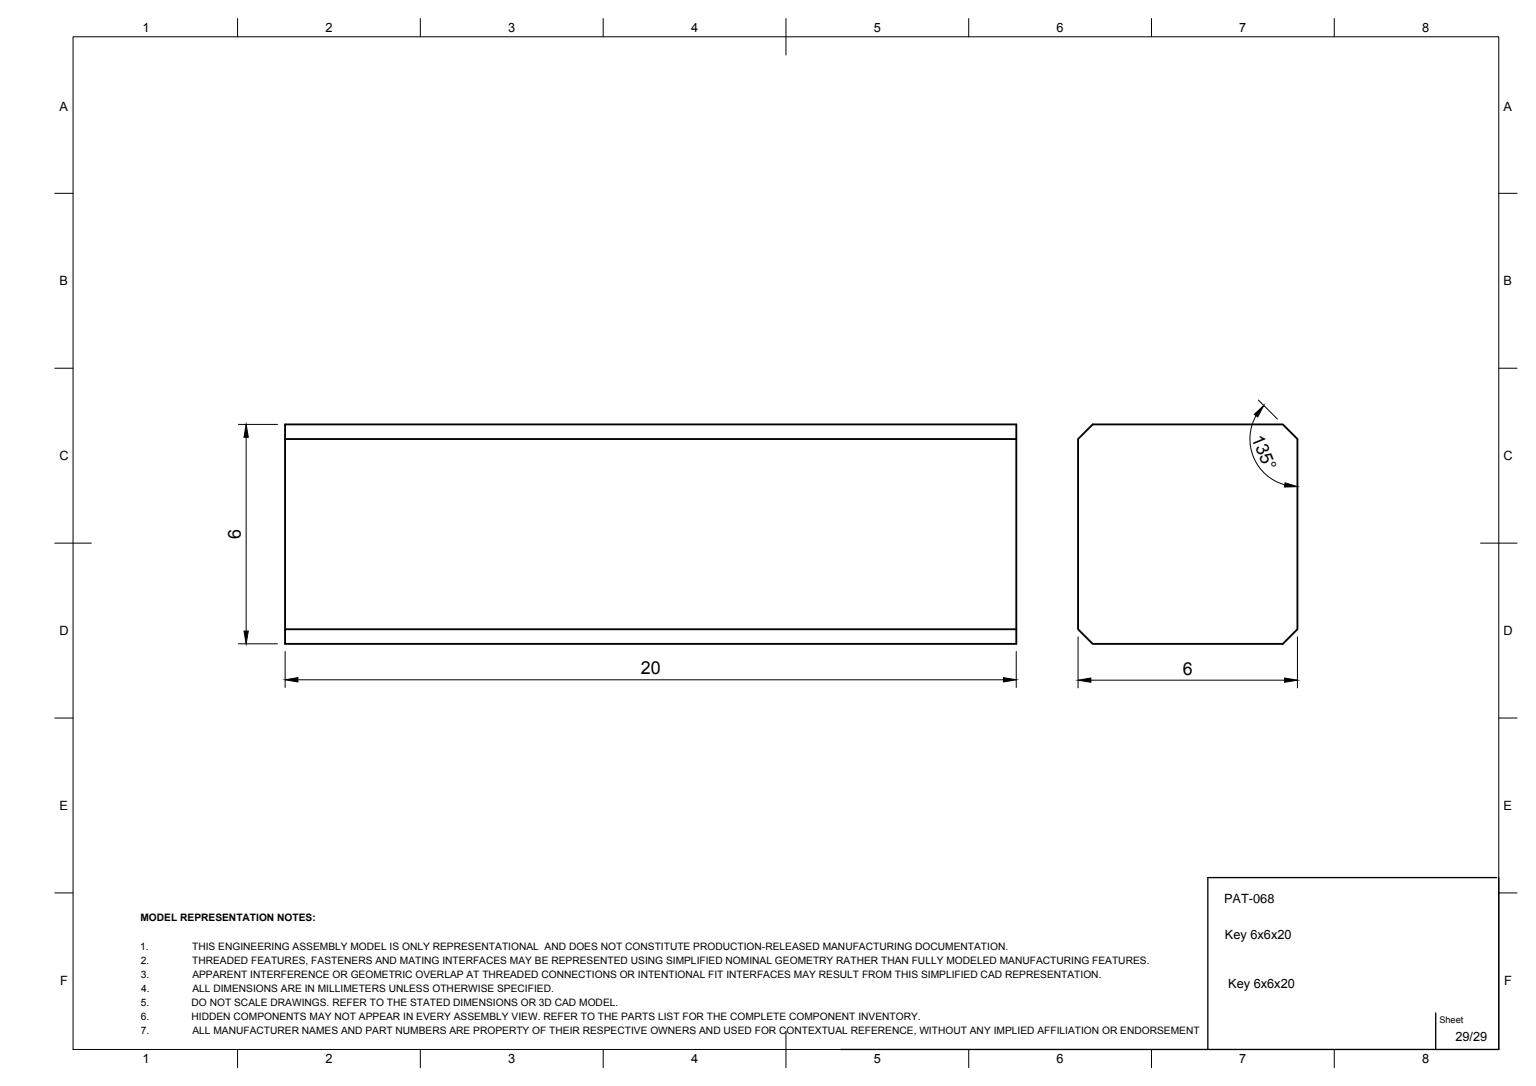
ISO-10303-21;
HEADER;
/* Generated by software containing ST-Developer
 * from STEP Tools, Inc. (www.steptools.com) 
 */

FILE_DESCRIPTION(
/* description */ ('Line shaft on three pillow blocks'),
/* implementation_level */ '2;1');

FILE_NAME(
/* name */ 'Key 6x6x20.step',
/* time_stamp */ '2026-10-27T10:49:19-07:00',
/* author */ (''),
/* organization */ (''),
/* preprocessor_version */ 'ST-DEVELOPER v20.2',
/* originating_system */ 'Autodesk Translation Framework v15.17.0.0',
/* authorisation */ '');

FILE_SCHEMA (('AUTOMOTIVE_DESIGN { 1 0 10303 214 3 1 1 }'));
ENDSEC;

DATA;
#10=MECHANICAL_DESIGN_GEOMETRIC_PRESENTATION_REPRESENTATION('',(#363),#8377);
#308=SHAPE_REPRESENTATION_RELATIONSHIP('SRR','None',#8525,#335);
#335=ADVANCED_BREP_SHAPE_REPRESENTATION('',(#389),#8374);
#363=STYLED_ITEM('',(#8718),#389);
#389=MANIFOLD_SOLID_BREP('Body1',#4351);
#624=PLANE('',#5078);
#625=PLANE('',#5079);
#626=PLANE('',#5080);
#627=PLANE('',#5081);
#628=PLANE('',#5082);
#629=PLANE('',#5083);
#630=PLANE('',#5084);
#631=PLANE('',#5085);
#632=PLANE('',#5086);
#633=PLANE('',#5087);
#867=FACE_OUTER_BOUND('',#1214,.T.);
#868=FACE_OUTER_BOUND('',#1215,.T.);
#869=FACE_OUTER_BOUND('',#1216,.T.);
#870=FACE_OUTER_BOUND('',#1217,.T.);
#871=FACE_OUTER_BOUND('',#1218,.T.);
#872=FACE_OUTER_BOUND('',#1219,.T.);
#873=FACE_OUTER_BOUND('',#1220,.T.);
#874=FACE_OUTER_BOUND('',#1221,.T.);
#875=FACE_OUTER_BOUND('',#1222,.T.);
#876=FACE_OUTER_BOUND('',#1223,.T.);
#1214=EDGE_LOOP('',(#3839,#3840,#3841,#3842,#3843,#3844,#3845,#3846));
#1215=EDGE_LOOP('',(#3847,#3848,#3849,#3850));
#1216=EDGE_LOOP('',(#3851,#3852,#3853,#3854));
#1217=EDGE_LOOP('',(#3855,#3856,#3857,#3858));
#1218=EDGE_LOOP('',(#3859,#3860,#3861,#3862));
#1219=EDGE_LOOP('',(#3863,#3864,#3865,#3866,#3867,#3868,#3869,#3870));
#1220=EDGE_LOOP('',(#3871,#3872,#3873,#3874));
#1221=EDGE_LOOP('',(#3875,#3876,#3877,#3878));
#1222=EDGE_LOOP('',(#3879,#3880,#3881,#3882));
#1223=EDGE_LOOP('',(#3883,#3884,#3885,#3886));
#1513=LINE('',#8126,#1840);
#1514=LINE('',#8128,#1841);
#1515=LINE('',#8130,#1842);
#1516=LINE('',#8132,#1843);
#1517=LINE('',#8134,#1844);
#1518=LINE('',#8136,#1845);
#1519=LINE('',#8138,#1846);
#1520=LINE('',#8139,#1847);
#1521=LINE('',#8142,#1848);
#1522=LINE('',#8144,#1849);
#1523=LINE('',#8145,#1850);
#1524=LINE('',#8148,#1851);
#1525=LINE('',#8149,#1852);
#1526=LINE('',#8152,#1853);
#1527=LINE('',#8153,#1854);
#1528=LINE('',#8156,#1855);
#1529=LINE('',#8157,#1856);
#1530=LINE('',#8161,#1857);
#1531=LINE('',#8162,#1858);
#1532=LINE('',#8164,#1859);
#1533=LINE('',#8165,#1860);
#1534=LINE('',#8167,#1861);
#1535=LINE('',#8169,#1862);
#1536=LINE('',#8171,#1863);
#1840=VECTOR('',#6258,1.);
#1841=VECTOR('',#6259,1.);
#1842=VECTOR('',#6260,1.);
#1843=VECTOR('',#6261,1.);
#1844=VECTOR('',#6262,1.);
#1845=VECTOR('',#6263,1.);
#1846=VECTOR('',#6264,1.);
#1847=VECTOR('',#6265,1.);
#1848=VECTOR('',#6268,1.);
#1849=VECTOR('',#6269,1.);
#1850=VECTOR('',#6270,1.);
#1851=VECTOR('',#6273,1.);
#1852=VECTOR('',#6274,1.);
#1853=VECTOR('',#6277,1.);
#1854=VECTOR('',#6278,1.);
#1855=VECTOR('',#6281,1.);
#1856=VECTOR('',#6282,1.);
#1857=VECTOR('',#6285,1.);
#1858=VECTOR('',#6286,1.);
#1859=VECTOR('',#6287,1.);
#1860=VECTOR('',#6288,1.);
#1861=VECTOR('',#6291,1.);
#1862=VECTOR('',#6294,1.);
#1863=VECTOR('',#6297,1.);
#2371=VERTEX_POINT('',#8124);
#2372=VERTEX_POINT('',#8125);
#2373=VERTEX_POINT('',#8127);
#2374=VERTEX_POINT('',#8129);
#2375=VERTEX_POINT('',#8131);
#2376=VERTEX_POINT('',#8133);
#2377=VERTEX_POINT('',#8135);
#2378=VERTEX_POINT('',#8137);
#2379=VERTEX_POINT('',#8141);
#2380=VERTEX_POINT('',#8143);
#2381=VERTEX_POINT('',#8147);
#2382=VERTEX_POINT('',#8151);
#2383=VERTEX_POINT('',#8155);
#2384=VERTEX_POINT('',#8159);
#2385=VERTEX_POINT('',#8160);
#2386=VERTEX_POINT('',#8163);
#2868=EDGE_CURVE('',#2371,#2372,#1513,.T.);
#2869=EDGE_CURVE('',#2373,#2371,#1514,.T.);
#2870=EDGE_CURVE('',#2374,#2373,#1515,.T.);
#2871=EDGE_CURVE('',#2375,#2374,#1516,.T.);
#2872=EDGE_CURVE('',#2376,#2375,#1517,.T.);
#2873=EDGE_CURVE('',#2377,#2376,#1518,.T.);
#2874=EDGE_CURVE('',#2378,#2377,#1519,.T.);
#2875=EDGE_CURVE('',#2372,#2378,#1520,.T.);
#2876=EDGE_CURVE('',#2375,#2379,#1521,.T.);
#2877=EDGE_CURVE('',#2379,#2380,#1522,.T.);
#2878=EDGE_CURVE('',#2380,#2376,#1523,.T.);
#2879=EDGE_CURVE('',#2381,#2374,#1524,.T.);
#2880=EDGE_CURVE('',#2381,#2379,#1525,.T.);
#2881=EDGE_CURVE('',#2373,#2382,#1526,.T.);
#2882=EDGE_CURVE('',#2382,#2381,#1527,.T.);
#2883=EDGE_CURVE('',#2383,#2371,#1528,.T.);
#2884=EDGE_CURVE('',#2383,#2382,#1529,.T.);
#2885=EDGE_CURVE('',#2384,#2385,#1530,.T.);
#2886=EDGE_CURVE('',#2380,#2384,#1531,.T.);
#2887=EDGE_CURVE('',#2386,#2383,#1532,.T.);
#2888=EDGE_CURVE('',#2385,#2386,#1533,.T.);
#2889=EDGE_CURVE('',#2377,#2384,#1534,.T.);
#2890=EDGE_CURVE('',#2372,#2386,#1535,.T.);
#2891=EDGE_CURVE('',#2385,#2378,#1536,.T.);
#3839=ORIENTED_EDGE('',*,*,#2868,.F.);
#3840=ORIENTED_EDGE('',*,*,#2869,.F.);
#3841=ORIENTED_EDGE('',*,*,#2870,.F.);
#3842=ORIENTED_EDGE('',*,*,#2871,.F.);
#3843=ORIENTED_EDGE('',*,*,#2872,.F.);
#3844=ORIENTED_EDGE('',*,*,#2873,.F.);
#3845=ORIENTED_EDGE('',*,*,#2874,.F.);
#3846=ORIENTED_EDGE('',*,*,#2875,.F.);
#3847=ORIENTED_EDGE('',*,*,#2872,.T.);
#3848=ORIENTED_EDGE('',*,*,#2876,.T.);
#3849=ORIENTED_EDGE('',*,*,#2877,.T.);
#3850=ORIENTED_EDGE('',*,*,#2878,.T.);
#3851=ORIENTED_EDGE('',*,*,#2871,.T.);
#3852=ORIENTED_EDGE('',*,*,#2879,.F.);
#3853=ORIENTED_EDGE('',*,*,#2880,.T.);
#3854=ORIENTED_EDGE('',*,*,#2876,.F.);
#3855=ORIENTED_EDGE('',*,*,#2870,.T.);
#3856=ORIENTED_EDGE('',*,*,#2881,.T.);
#3857=ORIENTED_EDGE('',*,*,#2882,.T.);
#3858=ORIENTED_EDGE('',*,*,#2879,.T.);
#3859=ORIENTED_EDGE('',*,*,#2869,.T.);
#3860=ORIENTED_EDGE('',*,*,#2883,.F.);
#3861=ORIENTED_EDGE('',*,*,#2884,.T.);
#3862=ORIENTED_EDGE('',*,*,#2881,.F.);
#3863=ORIENTED_EDGE('',*,*,#2885,.F.);
#3864=ORIENTED_EDGE('',*,*,#2886,.F.);
#3865=ORIENTED_EDGE('',*,*,#2877,.F.);
#3866=ORIENTED_EDGE('',*,*,#2880,.F.);
#3867=ORIENTED_EDGE('',*,*,#2882,.F.);
#3868=ORIENTED_EDGE('',*,*,#2884,.F.);
#3869=ORIENTED_EDGE('',*,*,#2887,.F.);
#3870=ORIENTED_EDGE('',*,*,#2888,.F.);
#3871=ORIENTED_EDGE('',*,*,#2873,.T.);
#3872=ORIENTED_EDGE('',*,*,#2878,.F.);
#3873=ORIENTED_EDGE('',*,*,#2886,.T.);
#3874=ORIENTED_EDGE('',*,*,#2889,.F.);
#3875=ORIENTED_EDGE('',*,*,#2868,.T.);
#3876=ORIENTED_EDGE('',*,*,#2890,.T.);
#3877=ORIENTED_EDGE('',*,*,#2887,.T.);
#3878=ORIENTED_EDGE('',*,*,#2883,.T.);
#3879=ORIENTED_EDGE('',*,*,#2874,.T.);
#3880=ORIENTED_EDGE('',*,*,#2889,.T.);
#3881=ORIENTED_EDGE('',*,*,#2885,.T.);
#3882=ORIENTED_EDGE('',*,*,#2891,.T.);
#3883=ORIENTED_EDGE('',*,*,#2875,.T.);
#3884=ORIENTED_EDGE('',*,*,#2891,.F.);
#3885=ORIENTED_EDGE('',*,*,#2888,.T.);
#3886=ORIENTED_EDGE('',*,*,#2890,.F.);
#4285=ADVANCED_FACE('',(#867),#624,.F.);
#4286=ADVANCED_FACE('',(#868),#625,.T.);
#4287=ADVANCED_FACE('',(#869),#626,.T.);
#4288=ADVANCED_FACE('',(#870),#627,.T.);
#4289=ADVANCED_FACE('',(#871),#628,.T.);
#4290=ADVANCED_FACE('',(#872),#629,.T.);
#4291=ADVANCED_FACE('',(#873),#630,.F.);
#4292=ADVANCED_FACE('',(#874),#631,.T.);
#4293=ADVANCED_FACE('',(#875),#632,.T.);
#4294=ADVANCED_FACE('',(#876),#633,.T.);
#4351=CLOSED_SHELL('',(#4285,#4286,#4287,#4288,#4289,#4290,#4291,#4292,
#4293,#4294));
#5077=AXIS2_PLACEMENT_3D('',#8122,#6254,#6255);
#5078=AXIS2_PLACEMENT_3D('',#8123,#6256,#6257);
#5079=AXIS2_PLACEMENT_3D('',#8140,#6266,#6267);
#5080=AXIS2_PLACEMENT_3D('',#8146,#6271,#6272);
#5081=AXIS2_PLACEMENT_3D('',#8150,#6275,#6276);
#5082=AXIS2_PLACEMENT_3D('',#8154,#6279,#6280);
#5083=AXIS2_PLACEMENT_3D('',#8158,#6283,#6284);
#5084=AXIS2_PLACEMENT_3D('',#8166,#6289,#6290);
#5085=AXIS2_PLACEMENT_3D('',#8168,#6292,#6293);
#5086=AXIS2_PLACEMENT_3D('',#8170,#6295,#6296);
#5087=AXIS2_PLACEMENT_3D('',#8172,#6298,#6299);
#6254=DIRECTION('axis',(0.,0.,1.));
#6255=DIRECTION('refdir',(1.,0.,0.));
#6256=DIRECTION('center_axis',(1.,0.,0.));
#6257=DIRECTION('ref_axis',(0.,0.,-1.));
#6258=DIRECTION('',(0.,-0.707106781186547,-0.707106781186548));
#6259=DIRECTION('',(0.,-1.,0.));
#6260=DIRECTION('',(0.,-0.707106781186547,0.707106781186548));
#6261=DIRECTION('',(0.,0.,1.));
#6262=DIRECTION('',(0.,0.707106781186547,0.707106781186548));
#6263=DIRECTION('',(0.,1.,0.));
#6264=DIRECTION('',(0.,0.707106781186547,-0.707106781186548));
#6265=DIRECTION('',(0.,0.,-1.));
#6266=DIRECTION('center_axis',(0.,0.707106781186548,-0.707106781186547));
#6267=DIRECTION('ref_axis',(-1.,0.,0.));
#6268=DIRECTION('',(1.,0.,0.));
#6269=DIRECTION('',(0.,-0.707106781186547,-0.707106781186548));
#6270=DIRECTION('',(-1.,0.,0.));
#6271=DIRECTION('center_axis',(0.,1.,0.));
#6272=DIRECTION('ref_axis',(-1.,0.,0.));
#6273=DIRECTION('',(-1.,0.,0.));
#6274=DIRECTION('',(0.,0.,-1.));
#6275=DIRECTION('center_axis',(0.,0.707106781186548,0.707106781186547));
#6276=DIRECTION('ref_axis',(1.,0.,0.));
#6277=DIRECTION('',(1.,0.,0.));
#6278=DIRECTION('',(0.,0.707106781186547,-0.707106781186548));
#6279=DIRECTION('center_axis',(0.,0.,1.));
#6280=DIRECTION('ref_axis',(1.,0.,0.));
#6281=DIRECTION('',(-1.,0.,0.));
#6282=DIRECTION('',(0.,1.,0.));
#6283=DIRECTION('center_axis',(1.,0.,0.));
#6284=DIRECTION('ref_axis',(0.,0.,-1.));
#6285=DIRECTION('',(0.,-0.707106781186547,0.707106781186548));
#6286=DIRECTION('',(0.,-1.,0.));
#6287=DIRECTION('',(0.,0.707106781186547,0.707106781186548));
#6288=DIRECTION('',(0.,0.,1.));
#6289=DIRECTION('center_axis',(0.,0.,1.));
#6290=DIRECTION('ref_axis',(1.,0.,0.));
#6291=DIRECTION('',(1.,0.,0.));
#6292=DIRECTION('center_axis',(0.,-0.707106781186548,0.707106781186547));
#6293=DIRECTION('ref_axis',(1.,0.,0.));
#6294=DIRECTION('',(1.,0.,0.));
#6295=DIRECTION('center_axis',(0.,-0.707106781186548,-0.707106781186547));
#6296=DIRECTION('ref_axis',(-1.,0.,0.));
#6297=DIRECTION('',(-1.,0.,0.));
#6298=DIRECTION('center_axis',(0.,-1.,0.));
#6299=DIRECTION('ref_axis',(1.,0.,0.));
#8122=CARTESIAN_POINT('',(0.,0.,0.));
#8123=CARTESIAN_POINT('Origin',(-1.,0.,0.35));
#8124=CARTESIAN_POINT('',(-1.,-0.26,0.6));
#8125=CARTESIAN_POINT('',(-1.,-0.3,0.56));
#8126=CARTESIAN_POINT('',(-1.,-0.2675,0.5925));
#8127=CARTESIAN_POINT('',(-1.,0.26,0.6));
#8128=CARTESIAN_POINT('',(-1.,0.,0.6));
#8129=CARTESIAN_POINT('',(-1.,0.3,0.56));
#8130=CARTESIAN_POINT('',(-1.,0.2675,0.5925));
#8131=CARTESIAN_POINT('',(-1.,0.3,0.04));
#8132=CARTESIAN_POINT('',(-1.,0.3,0.175));
#8133=CARTESIAN_POINT('',(-1.,0.26,0.));
#8134=CARTESIAN_POINT('',(-1.,0.2925,0.0325));
#8135=CARTESIAN_POINT('',(-1.,-0.26,0.));
#8136=CARTESIAN_POINT('',(-1.,0.,0.));
#8137=CARTESIAN_POINT('',(-1.,-0.3,0.04));
#8138=CARTESIAN_POINT('',(-1.,-0.2925,0.0325));
#8139=CARTESIAN_POINT('',(-1.,-0.3,0.175));
#8140=CARTESIAN_POINT('Origin',(0.75,0.28,0.02));
#8141=CARTESIAN_POINT('',(1.,0.3,0.04));
#8142=CARTESIAN_POINT('',(0.75,0.3,0.04));
#8143=CARTESIAN_POINT('',(1.,0.26,0.));
#8144=CARTESIAN_POINT('',(1.,0.2925,0.0325));
#8145=CARTESIAN_POINT('',(0.75,0.26,0.));
#8146=CARTESIAN_POINT('Origin',(1.5,0.3,0.));
#8147=CARTESIAN_POINT('',(1.,0.3,0.56));
#8148=CARTESIAN_POINT('',(0.75,0.3,0.56));
#8149=CARTESIAN_POINT('',(1.,0.3,0.175));
#8150=CARTESIAN_POINT('Origin',(0.75,0.28,0.58));
#8151=CARTESIAN_POINT('',(1.,0.26,0.6));
#8152=CARTESIAN_POINT('',(0.75,0.26,0.6));
#8153=CARTESIAN_POINT('',(1.,0.2675,0.5925));
#8154=CARTESIAN_POINT('Origin',(0.,0.,0.6));
#8155=CARTESIAN_POINT('',(1.,-0.26,0.6));
#8156=CARTESIAN_POINT('',(-0.75,-0.26,0.6));
#8157=CARTESIAN_POINT('',(1.,0.,0.6));
#8158=CARTESIAN_POINT('Origin',(1.,0.,0.35));
#8159=CARTESIAN_POINT('',(1.,-0.26,0.));
#8160=CARTESIAN_POINT('',(1.,-0.3,0.04));
#8161=CARTESIAN_POINT('',(1.,-0.2925,0.0325));
#8162=CARTESIAN_POINT('',(1.,0.,0.));
#8163=CARTESIAN_POINT('',(1.,-0.3,0.56));
#8164=CARTESIAN_POINT('',(1.,-0.2675,0.5925));
#8165=CARTESIAN_POINT('',(1.,-0.3,0.175));
#8166=CARTESIAN_POINT('Origin',(0.,0.,0.));
#8167=CARTESIAN_POINT('',(-0.75,-0.26,0.));
#8168=CARTESIAN_POINT('Origin',(-0.75,-0.28,0.58));
#8169=CARTESIAN_POINT('',(-0.75,-0.3,0.56));
#8170=CARTESIAN_POINT('Origin',(-0.75,-0.28,0.02));
#8171=CARTESIAN_POINT('',(-0.75,-0.3,0.04));
#8172=CARTESIAN_POINT('Origin',(-1.5,-0.3,0.));
#8342=UNCERTAINTY_MEASURE_WITH_UNIT(LENGTH_MEASURE(0.001),#8378,
'DISTANCE_ACCURACY_VALUE',
'Maximum model space distance between geometric entities at asserted c
onnectivities');
#8345=UNCERTAINTY_MEASURE_WITH_UNIT(LENGTH_MEASURE(0.001),#8378,
'DISTANCE_ACCURACY_VALUE',
'Maximum model space distance between geometric entities at asserted c
onnectivities');
#8374=(
GEOMETRIC_REPRESENTATION_CONTEXT(3)
GLOBAL_UNCERTAINTY_ASSIGNED_CONTEXT((#8342))
GLOBAL_UNIT_ASSIGNED_CONTEXT((#8378,#8380,#8381))
REPRESENTATION_CONTEXT('','3D')
);
#8377=(
GEOMETRIC_REPRESENTATION_CONTEXT(3)
GLOBAL_UNCERTAINTY_ASSIGNED_CONTEXT((#8345))
GLOBAL_UNIT_ASSIGNED_CONTEXT((#8378,#8380,#8381))
REPRESENTATION_CONTEXT('','3D')
);
#8378=(
LENGTH_UNIT()
NAMED_UNIT(*)
SI_UNIT(.CENTI.,.METRE.)
);
#8380=(
NAMED_UNIT(*)
PLANE_ANGLE_UNIT()
SI_UNIT($,.RADIAN.)
);
#8381=(
NAMED_UNIT(*)
SI_UNIT($,.STERADIAN.)
SOLID_ANGLE_UNIT()
);
#8410=SHAPE_DEFINITION_REPRESENTATION(#8477,#8525);
#8477=PRODUCT_DEFINITION_SHAPE('',$,#8557);
#8525=SHAPE_REPRESENTATION('',(#5077),#8374);
#8528=PRODUCT_DEFINITION_CONTEXT('part definition',#8623,'design');
#8557=PRODUCT_DEFINITION('Key 6x6x20','Key 6x6x20',#8588,#8528);
#8588=PRODUCT_DEFINITION_FORMATION('',$,#8653);
#8623=APPLICATION_CONTEXT(
'Core Data for Automotive Mechanical Design Process');
#8624=PRODUCT_CONTEXT('part definition',#8623,'mechanical');
#8653=PRODUCT('Key 6x6x20','Key 6x6x20','Key 6x6x20',(#8624));
#8712=COLOUR_RGB('Grey',0.48,0.52,0.57);
#8713=FILL_AREA_STYLE_COLOUR('',#8712);
#8714=FILL_AREA_STYLE('',(#8713));
#8715=SURFACE_STYLE_FILL_AREA(#8714);
#8716=SURFACE_SIDE_STYLE('',(#8715));
#8717=SURFACE_STYLE_USAGE(.BOTH.,#8716);
#8718=PRESENTATION_STYLE_ASSIGNMENT((#8717));
ENDSEC;
END-ISO-10303-21;
